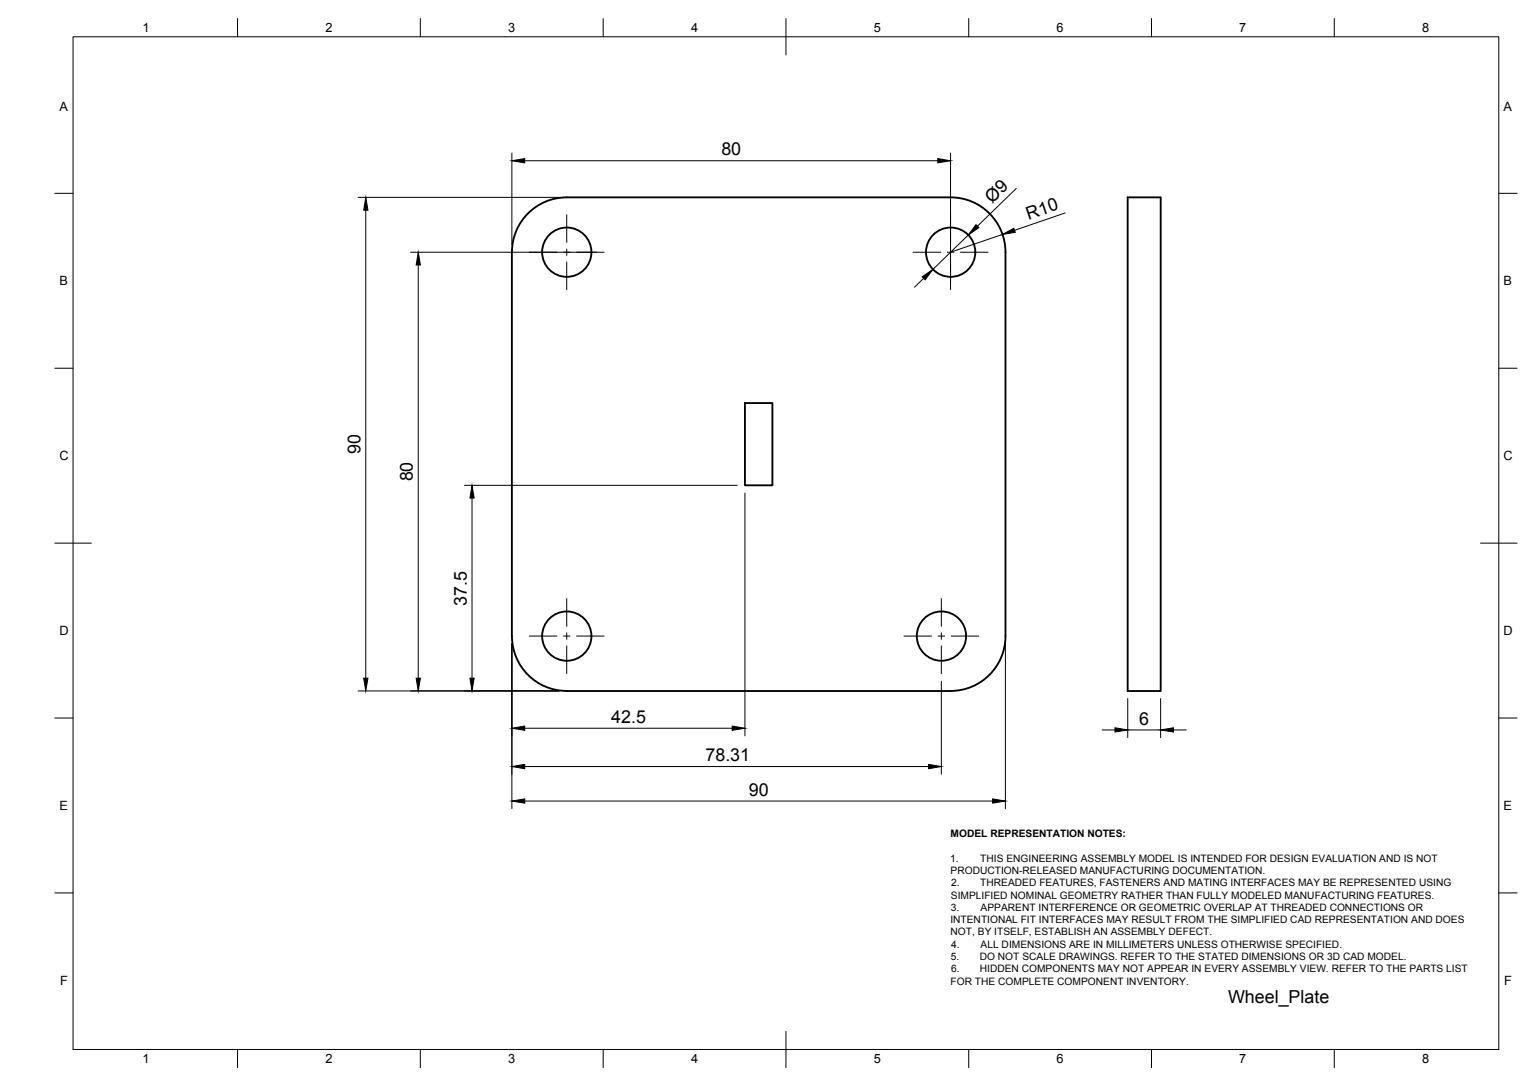
ISO-10303-21;
HEADER;
/* Generated by software containing ST-Developer
 * from STEP Tools, Inc. (www.steptools.com) 
 */

FILE_DESCRIPTION(
/* description */ ('Wheel Holder-Mirrored'),
/* implementation_level */ '2;1');

FILE_NAME(
/* name */ 'Wheel_Plate.step',
/* time_stamp */ '2026-10-07T09:01:46-07:00',
/* author */ (''),
/* organization */ (''),
/* preprocessor_version */ 'ST-DEVELOPER v20.2',
/* originating_system */ 'Autodesk Translation Framework v15.15.0.0',
/* authorisation */ '');

FILE_SCHEMA (('AUTOMOTIVE_DESIGN { 1 0 10303 214 3 1 1 }'));
ENDSEC;

DATA;
#10=MECHANICAL_DESIGN_GEOMETRIC_PRESENTATION_REPRESENTATION('',(#200),#3832);
#188=SHAPE_REPRESENTATION_RELATIONSHIP('SRR','None',#3865,#194);
#194=ADVANCED_BREP_SHAPE_REPRESENTATION('',(#206),#3828);
#200=STYLED_ITEM('',(#3904),#206);
#206=MANIFOLD_SOLID_BREP('Body1',#1785);
#214=FACE_BOUND('',#393,.T.);
#215=FACE_BOUND('',#394,.T.);
#216=FACE_BOUND('',#395,.T.);
#217=FACE_BOUND('',#396,.T.);
#218=FACE_BOUND('',#397,.T.);
#219=FACE_BOUND('',#399,.T.);
#220=FACE_BOUND('',#400,.T.);
#221=FACE_BOUND('',#401,.T.);
#222=FACE_BOUND('',#402,.T.);
#223=FACE_BOUND('',#403,.T.);
#233=PLANE('',#1881);
#234=PLANE('',#1890);
#235=PLANE('',#1899);
#236=PLANE('',#1901);
#237=PLANE('',#1903);
#238=PLANE('',#1905);
#239=PLANE('',#1911);
#240=PLANE('',#1912);
#241=PLANE('',#1913);
#242=PLANE('',#1914);
#284=FACE_OUTER_BOUND('',#392,.T.);
#285=FACE_OUTER_BOUND('',#398,.T.);
#286=FACE_OUTER_BOUND('',#404,.T.);
#287=FACE_OUTER_BOUND('',#405,.T.);
#288=FACE_OUTER_BOUND('',#406,.T.);
#289=FACE_OUTER_BOUND('',#407,.T.);
#290=FACE_OUTER_BOUND('',#408,.T.);
#291=FACE_OUTER_BOUND('',#409,.T.);
#292=FACE_OUTER_BOUND('',#410,.T.);
#293=FACE_OUTER_BOUND('',#411,.T.);
#294=FACE_OUTER_BOUND('',#412,.T.);
#295=FACE_OUTER_BOUND('',#413,.T.);
#296=FACE_OUTER_BOUND('',#414,.T.);
#297=FACE_OUTER_BOUND('',#415,.T.);
#298=FACE_OUTER_BOUND('',#416,.T.);
#299=FACE_OUTER_BOUND('',#417,.T.);
#300=FACE_OUTER_BOUND('',#418,.T.);
#301=FACE_OUTER_BOUND('',#419,.T.);
#392=EDGE_LOOP('',(#1183,#1184,#1185,#1186,#1187,#1188,#1189,#1190));
#393=EDGE_LOOP('',(#1191,#1192,#1193,#1194));
#394=EDGE_LOOP('',(#1195));
#395=EDGE_LOOP('',(#1196));
#396=EDGE_LOOP('',(#1197));
#397=EDGE_LOOP('',(#1198));
#398=EDGE_LOOP('',(#1199,#1200,#1201,#1202,#1203,#1204,#1205,#1206));
#399=EDGE_LOOP('',(#1207));
#400=EDGE_LOOP('',(#1208));
#401=EDGE_LOOP('',(#1209));
#402=EDGE_LOOP('',(#1210));
#403=EDGE_LOOP('',(#1211,#1212,#1213,#1214));
#404=EDGE_LOOP('',(#1215,#1216,#1217,#1218));
#405=EDGE_LOOP('',(#1219,#1220,#1221,#1222));
#406=EDGE_LOOP('',(#1223,#1224,#1225,#1226));
#407=EDGE_LOOP('',(#1227,#1228,#1229,#1230));
#408=EDGE_LOOP('',(#1231,#1232,#1233,#1234));
#409=EDGE_LOOP('',(#1235,#1236,#1237,#1238));
#410=EDGE_LOOP('',(#1239,#1240,#1241,#1242));
#411=EDGE_LOOP('',(#1243,#1244,#1245,#1246));
#412=EDGE_LOOP('',(#1247,#1248,#1249,#1250));
#413=EDGE_LOOP('',(#1251,#1252,#1253,#1254));
#414=EDGE_LOOP('',(#1255,#1256,#1257,#1258));
#415=EDGE_LOOP('',(#1259,#1260,#1261,#1262));
#416=EDGE_LOOP('',(#1263,#1264,#1265,#1266));
#417=EDGE_LOOP('',(#1267,#1268,#1269,#1270));
#418=EDGE_LOOP('',(#1271,#1272,#1273,#1274));
#419=EDGE_LOOP('',(#1275,#1276,#1277,#1278));
#503=LINE('',#2568,#596);
#504=LINE('',#2572,#597);
#505=LINE('',#2576,#598);
#506=LINE('',#2580,#599);
#507=LINE('',#2584,#600);
#508=LINE('',#2586,#601);
#509=LINE('',#2588,#602);
#510=LINE('',#2589,#603);
#511=LINE('',#2601,#604);
#512=LINE('',#2605,#605);
#513=LINE('',#2609,#606);
#514=LINE('',#2613,#607);
#515=LINE('',#2625,#608);
#516=LINE('',#2627,#609);
#517=LINE('',#2629,#610);
#518=LINE('',#2630,#611);
#519=LINE('',#2632,#612);
#520=LINE('',#2633,#613);
#521=LINE('',#2635,#614);
#522=LINE('',#2637,#615);
#523=LINE('',#2639,#616);
#524=LINE('',#2641,#617);
#525=LINE('',#2643,#618);
#526=LINE('',#2645,#619);
#527=LINE('',#2647,#620);
#528=LINE('',#2649,#621);
#529=LINE('',#2651,#622);
#530=LINE('',#2653,#623);
#531=LINE('',#2656,#624);
#532=LINE('',#2657,#625);
#533=LINE('',#2659,#626);
#534=LINE('',#2661,#627);
#596=VECTOR('',#2105,1.);
#597=VECTOR('',#2108,1.);
#598=VECTOR('',#2111,1.);
#599=VECTOR('',#2114,1.);
#600=VECTOR('',#2117,1.);
#601=VECTOR('',#2118,1.);
#602=VECTOR('',#2119,1.);
#603=VECTOR('',#2120,1.);
#604=VECTOR('',#2131,1.);
#605=VECTOR('',#2134,1.);
#606=VECTOR('',#2137,1.);
#607=VECTOR('',#2140,1.);
#608=VECTOR('',#2151,1.);
#609=VECTOR('',#2152,1.);
#610=VECTOR('',#2153,1.);
#611=VECTOR('',#2154,1.);
#612=VECTOR('',#2157,1.);
#613=VECTOR('',#2158,1.);
#614=VECTOR('',#2161,1.);
#615=VECTOR('',#2164,1.);
#616=VECTOR('',#2167,1.);
#617=VECTOR('',#2170,1.);
#618=VECTOR('',#2173,1.);
#619=VECTOR('',#2176,1.);
#620=VECTOR('',#2179,0.0045);
#621=VECTOR('',#2182,0.0045);
#622=VECTOR('',#2185,0.0045);
#623=VECTOR('',#2188,0.0045);
#624=VECTOR('',#2193,1.);
#625=VECTOR('',#2194,1.);
#626=VECTOR('',#2197,1.);
#627=VECTOR('',#2200,1.);
#694=CIRCLE('',#1882,0.01);
#695=CIRCLE('',#1883,0.0100000000000001);
#696=CIRCLE('',#1884,0.0100000000000001);
#697=CIRCLE('',#1885,0.01);
#698=CIRCLE('',#1886,0.0045);
#699=CIRCLE('',#1887,0.0045);
#700=CIRCLE('',#1888,0.0045);
#701=CIRCLE('',#1889,0.0045);
#702=CIRCLE('',#1891,0.01);
#703=CIRCLE('',#1892,0.0100000000000001);
#704=CIRCLE('',#1893,0.0100000000000001);
#705=CIRCLE('',#1894,0.01);
#706=CIRCLE('',#1895,0.0045);
#707=CIRCLE('',#1896,0.0045);
#708=CIRCLE('',#1897,0.0045);
#709=CIRCLE('',#1898,0.0045);
#756=VERTEX_POINT('',#2566);
#757=VERTEX_POINT('',#2567);
#758=VERTEX_POINT('',#2569);
#759=VERTEX_POINT('',#2571);
#760=VERTEX_POINT('',#2573);
#761=VERTEX_POINT('',#2575);
#762=VERTEX_POINT('',#2577);
#763=VERTEX_POINT('',#2579);
#764=VERTEX_POINT('',#2582);
#765=VERTEX_POINT('',#2583);
#766=VERTEX_POINT('',#2585);
#767=VERTEX_POINT('',#2587);
#768=VERTEX_POINT('',#2590);
#769=VERTEX_POINT('',#2592);
#770=VERTEX_POINT('',#2594);
#771=VERTEX_POINT('',#2596);
#772=VERTEX_POINT('',#2599);
#773=VERTEX_POINT('',#2600);
#774=VERTEX_POINT('',#2602);
#775=VERTEX_POINT('',#2604);
#776=VERTEX_POINT('',#2606);
#777=VERTEX_POINT('',#2608);
#778=VERTEX_POINT('',#2610);
#779=VERTEX_POINT('',#2612);
#780=VERTEX_POINT('',#2615);
#781=VERTEX_POINT('',#2617);
#782=VERTEX_POINT('',#2619);
#783=VERTEX_POINT('',#2621);
#784=VERTEX_POINT('',#2623);
#785=VERTEX_POINT('',#2624);
#786=VERTEX_POINT('',#2626);
#787=VERTEX_POINT('',#2628);
#918=EDGE_CURVE('',#756,#757,#503,.T.);
#919=EDGE_CURVE('',#758,#756,#694,.T.);
#920=EDGE_CURVE('',#758,#759,#504,.T.);
#921=EDGE_CURVE('',#760,#759,#695,.T.);
#922=EDGE_CURVE('',#760,#761,#505,.T.);
#923=EDGE_CURVE('',#762,#761,#696,.T.);
#924=EDGE_CURVE('',#763,#762,#506,.T.);
#925=EDGE_CURVE('',#757,#763,#697,.T.);
#926=EDGE_CURVE('',#764,#765,#507,.T.);
#927=EDGE_CURVE('',#765,#766,#508,.T.);
#928=EDGE_CURVE('',#767,#766,#509,.T.);
#929=EDGE_CURVE('',#764,#767,#510,.T.);
#930=EDGE_CURVE('',#768,#768,#698,.T.);
#931=EDGE_CURVE('',#769,#769,#699,.T.);
#932=EDGE_CURVE('',#770,#770,#700,.T.);
#933=EDGE_CURVE('',#771,#771,#701,.T.);
#934=EDGE_CURVE('',#772,#773,#511,.T.);
#935=EDGE_CURVE('',#773,#774,#702,.T.);
#936=EDGE_CURVE('',#774,#775,#512,.T.);
#937=EDGE_CURVE('',#775,#776,#703,.T.);
#938=EDGE_CURVE('',#777,#776,#513,.T.);
#939=EDGE_CURVE('',#777,#778,#704,.T.);
#940=EDGE_CURVE('',#779,#778,#514,.T.);
#941=EDGE_CURVE('',#779,#772,#705,.T.);
#942=EDGE_CURVE('',#780,#780,#706,.T.);
#943=EDGE_CURVE('',#781,#781,#707,.T.);
#944=EDGE_CURVE('',#782,#782,#708,.T.);
#945=EDGE_CURVE('',#783,#783,#709,.T.);
#946=EDGE_CURVE('',#784,#785,#515,.T.);
#947=EDGE_CURVE('',#786,#784,#516,.T.);
#948=EDGE_CURVE('',#786,#787,#517,.T.);
#949=EDGE_CURVE('',#787,#785,#518,.T.);
#950=EDGE_CURVE('',#756,#772,#519,.T.);
#951=EDGE_CURVE('',#757,#773,#520,.T.);
#952=EDGE_CURVE('',#763,#774,#521,.T.);
#953=EDGE_CURVE('',#762,#775,#522,.T.);
#954=EDGE_CURVE('',#761,#776,#523,.T.);
#955=EDGE_CURVE('',#760,#777,#524,.T.);
#956=EDGE_CURVE('',#759,#778,#525,.T.);
#957=EDGE_CURVE('',#758,#779,#526,.T.);
#958=EDGE_CURVE('',#771,#780,#527,.T.);
#959=EDGE_CURVE('',#770,#781,#528,.T.);
#960=EDGE_CURVE('',#769,#782,#529,.T.);
#961=EDGE_CURVE('',#768,#783,#530,.T.);
#962=EDGE_CURVE('',#765,#784,#531,.T.);
#963=EDGE_CURVE('',#766,#785,#532,.T.);
#964=EDGE_CURVE('',#767,#787,#533,.T.);
#965=EDGE_CURVE('',#764,#786,#534,.T.);
#1183=ORIENTED_EDGE('',*,*,#918,.F.);
#1184=ORIENTED_EDGE('',*,*,#919,.F.);
#1185=ORIENTED_EDGE('',*,*,#920,.T.);
#1186=ORIENTED_EDGE('',*,*,#921,.F.);
#1187=ORIENTED_EDGE('',*,*,#922,.T.);
#1188=ORIENTED_EDGE('',*,*,#923,.F.);
#1189=ORIENTED_EDGE('',*,*,#924,.F.);
#1190=ORIENTED_EDGE('',*,*,#925,.F.);
#1191=ORIENTED_EDGE('',*,*,#926,.T.);
#1192=ORIENTED_EDGE('',*,*,#927,.T.);
#1193=ORIENTED_EDGE('',*,*,#928,.F.);
#1194=ORIENTED_EDGE('',*,*,#929,.F.);
#1195=ORIENTED_EDGE('',*,*,#930,.T.);
#1196=ORIENTED_EDGE('',*,*,#931,.T.);
#1197=ORIENTED_EDGE('',*,*,#932,.T.);
#1198=ORIENTED_EDGE('',*,*,#933,.T.);
#1199=ORIENTED_EDGE('',*,*,#934,.T.);
#1200=ORIENTED_EDGE('',*,*,#935,.T.);
#1201=ORIENTED_EDGE('',*,*,#936,.T.);
#1202=ORIENTED_EDGE('',*,*,#937,.T.);
#1203=ORIENTED_EDGE('',*,*,#938,.F.);
#1204=ORIENTED_EDGE('',*,*,#939,.T.);
#1205=ORIENTED_EDGE('',*,*,#940,.F.);
#1206=ORIENTED_EDGE('',*,*,#941,.T.);
#1207=ORIENTED_EDGE('',*,*,#942,.F.);
#1208=ORIENTED_EDGE('',*,*,#943,.F.);
#1209=ORIENTED_EDGE('',*,*,#944,.F.);
#1210=ORIENTED_EDGE('',*,*,#945,.F.);
#1211=ORIENTED_EDGE('',*,*,#946,.F.);
#1212=ORIENTED_EDGE('',*,*,#947,.F.);
#1213=ORIENTED_EDGE('',*,*,#948,.T.);
#1214=ORIENTED_EDGE('',*,*,#949,.T.);
#1215=ORIENTED_EDGE('',*,*,#934,.F.);
#1216=ORIENTED_EDGE('',*,*,#950,.F.);
#1217=ORIENTED_EDGE('',*,*,#918,.T.);
#1218=ORIENTED_EDGE('',*,*,#951,.T.);
#1219=ORIENTED_EDGE('',*,*,#935,.F.);
#1220=ORIENTED_EDGE('',*,*,#951,.F.);
#1221=ORIENTED_EDGE('',*,*,#925,.T.);
#1222=ORIENTED_EDGE('',*,*,#952,.T.);
#1223=ORIENTED_EDGE('',*,*,#936,.F.);
#1224=ORIENTED_EDGE('',*,*,#952,.F.);
#1225=ORIENTED_EDGE('',*,*,#924,.T.);
#1226=ORIENTED_EDGE('',*,*,#953,.T.);
#1227=ORIENTED_EDGE('',*,*,#937,.F.);
#1228=ORIENTED_EDGE('',*,*,#953,.F.);
#1229=ORIENTED_EDGE('',*,*,#923,.T.);
#1230=ORIENTED_EDGE('',*,*,#954,.T.);
#1231=ORIENTED_EDGE('',*,*,#938,.T.);
#1232=ORIENTED_EDGE('',*,*,#954,.F.);
#1233=ORIENTED_EDGE('',*,*,#922,.F.);
#1234=ORIENTED_EDGE('',*,*,#955,.T.);
#1235=ORIENTED_EDGE('',*,*,#939,.F.);
#1236=ORIENTED_EDGE('',*,*,#955,.F.);
#1237=ORIENTED_EDGE('',*,*,#921,.T.);
#1238=ORIENTED_EDGE('',*,*,#956,.T.);
#1239=ORIENTED_EDGE('',*,*,#940,.T.);
#1240=ORIENTED_EDGE('',*,*,#956,.F.);
#1241=ORIENTED_EDGE('',*,*,#920,.F.);
#1242=ORIENTED_EDGE('',*,*,#957,.T.);
#1243=ORIENTED_EDGE('',*,*,#933,.F.);
#1244=ORIENTED_EDGE('',*,*,#958,.T.);
#1245=ORIENTED_EDGE('',*,*,#942,.T.);
#1246=ORIENTED_EDGE('',*,*,#958,.F.);
#1247=ORIENTED_EDGE('',*,*,#932,.F.);
#1248=ORIENTED_EDGE('',*,*,#959,.T.);
#1249=ORIENTED_EDGE('',*,*,#943,.T.);
#1250=ORIENTED_EDGE('',*,*,#959,.F.);
#1251=ORIENTED_EDGE('',*,*,#931,.F.);
#1252=ORIENTED_EDGE('',*,*,#960,.T.);
#1253=ORIENTED_EDGE('',*,*,#944,.T.);
#1254=ORIENTED_EDGE('',*,*,#960,.F.);
#1255=ORIENTED_EDGE('',*,*,#930,.F.);
#1256=ORIENTED_EDGE('',*,*,#961,.T.);
#1257=ORIENTED_EDGE('',*,*,#945,.T.);
#1258=ORIENTED_EDGE('',*,*,#961,.F.);
#1259=ORIENTED_EDGE('',*,*,#941,.F.);
#1260=ORIENTED_EDGE('',*,*,#957,.F.);
#1261=ORIENTED_EDGE('',*,*,#919,.T.);
#1262=ORIENTED_EDGE('',*,*,#950,.T.);
#1263=ORIENTED_EDGE('',*,*,#962,.T.);
#1264=ORIENTED_EDGE('',*,*,#946,.T.);
#1265=ORIENTED_EDGE('',*,*,#963,.F.);
#1266=ORIENTED_EDGE('',*,*,#927,.F.);
#1267=ORIENTED_EDGE('',*,*,#928,.T.);
#1268=ORIENTED_EDGE('',*,*,#963,.T.);
#1269=ORIENTED_EDGE('',*,*,#949,.F.);
#1270=ORIENTED_EDGE('',*,*,#964,.F.);
#1271=ORIENTED_EDGE('',*,*,#929,.T.);
#1272=ORIENTED_EDGE('',*,*,#964,.T.);
#1273=ORIENTED_EDGE('',*,*,#948,.F.);
#1274=ORIENTED_EDGE('',*,*,#965,.F.);
#1275=ORIENTED_EDGE('',*,*,#965,.T.);
#1276=ORIENTED_EDGE('',*,*,#947,.T.);
#1277=ORIENTED_EDGE('',*,*,#962,.F.);
#1278=ORIENTED_EDGE('',*,*,#926,.F.);
#1658=CYLINDRICAL_SURFACE('',#1900,0.01);
#1659=CYLINDRICAL_SURFACE('',#1902,0.0100000000000001);
#1660=CYLINDRICAL_SURFACE('',#1904,0.0100000000000001);
#1661=CYLINDRICAL_SURFACE('',#1906,0.0045);
#1662=CYLINDRICAL_SURFACE('',#1907,0.0045);
#1663=CYLINDRICAL_SURFACE('',#1908,0.0045);
#1664=CYLINDRICAL_SURFACE('',#1909,0.0045);
#1665=CYLINDRICAL_SURFACE('',#1910,0.01);
#1690=ADVANCED_FACE('',(#284,#214,#215,#216,#217,#218),#233,.T.);
#1691=ADVANCED_FACE('',(#285,#219,#220,#221,#222,#223),#234,.F.);
#1692=ADVANCED_FACE('',(#286),#235,.F.);
#1693=ADVANCED_FACE('',(#287),#1658,.T.);
#1694=ADVANCED_FACE('',(#288),#236,.F.);
#1695=ADVANCED_FACE('',(#289),#1659,.T.);
#1696=ADVANCED_FACE('',(#290),#237,.T.);
#1697=ADVANCED_FACE('',(#291),#1660,.T.);
#1698=ADVANCED_FACE('',(#292),#238,.T.);
#1699=ADVANCED_FACE('',(#293),#1661,.F.);
#1700=ADVANCED_FACE('',(#294),#1662,.F.);
#1701=ADVANCED_FACE('',(#295),#1663,.F.);
#1702=ADVANCED_FACE('',(#296),#1664,.F.);
#1703=ADVANCED_FACE('',(#297),#1665,.T.);
#1704=ADVANCED_FACE('',(#298),#239,.T.);
#1705=ADVANCED_FACE('',(#299),#240,.F.);
#1706=ADVANCED_FACE('',(#300),#241,.F.);
#1707=ADVANCED_FACE('',(#301),#242,.T.);
#1785=CLOSED_SHELL('',(#1690,#1691,#1692,#1693,#1694,#1695,#1696,#1697,
#1698,#1699,#1700,#1701,#1702,#1703,#1704,#1705,#1706,#1707));
#1880=AXIS2_PLACEMENT_3D('',#2564,#2101,#2102);
#1881=AXIS2_PLACEMENT_3D('',#2565,#2103,#2104);
#1882=AXIS2_PLACEMENT_3D('',#2570,#2106,#2107);
#1883=AXIS2_PLACEMENT_3D('',#2574,#2109,#2110);
#1884=AXIS2_PLACEMENT_3D('',#2578,#2112,#2113);
#1885=AXIS2_PLACEMENT_3D('',#2581,#2115,#2116);
#1886=AXIS2_PLACEMENT_3D('',#2591,#2121,#2122);
#1887=AXIS2_PLACEMENT_3D('',#2593,#2123,#2124);
#1888=AXIS2_PLACEMENT_3D('',#2595,#2125,#2126);
#1889=AXIS2_PLACEMENT_3D('',#2597,#2127,#2128);
#1890=AXIS2_PLACEMENT_3D('',#2598,#2129,#2130);
#1891=AXIS2_PLACEMENT_3D('',#2603,#2132,#2133);
#1892=AXIS2_PLACEMENT_3D('',#2607,#2135,#2136);
#1893=AXIS2_PLACEMENT_3D('',#2611,#2138,#2139);
#1894=AXIS2_PLACEMENT_3D('',#2614,#2141,#2142);
#1895=AXIS2_PLACEMENT_3D('',#2616,#2143,#2144);
#1896=AXIS2_PLACEMENT_3D('',#2618,#2145,#2146);
#1897=AXIS2_PLACEMENT_3D('',#2620,#2147,#2148);
#1898=AXIS2_PLACEMENT_3D('',#2622,#2149,#2150);
#1899=AXIS2_PLACEMENT_3D('',#2631,#2155,#2156);
#1900=AXIS2_PLACEMENT_3D('',#2634,#2159,#2160);
#1901=AXIS2_PLACEMENT_3D('',#2636,#2162,#2163);
#1902=AXIS2_PLACEMENT_3D('',#2638,#2165,#2166);
#1903=AXIS2_PLACEMENT_3D('',#2640,#2168,#2169);
#1904=AXIS2_PLACEMENT_3D('',#2642,#2171,#2172);
#1905=AXIS2_PLACEMENT_3D('',#2644,#2174,#2175);
#1906=AXIS2_PLACEMENT_3D('',#2646,#2177,#2178);
#1907=AXIS2_PLACEMENT_3D('',#2648,#2180,#2181);
#1908=AXIS2_PLACEMENT_3D('',#2650,#2183,#2184);
#1909=AXIS2_PLACEMENT_3D('',#2652,#2186,#2187);
#1910=AXIS2_PLACEMENT_3D('',#2654,#2189,#2190);
#1911=AXIS2_PLACEMENT_3D('',#2655,#2191,#2192);
#1912=AXIS2_PLACEMENT_3D('',#2658,#2195,#2196);
#1913=AXIS2_PLACEMENT_3D('',#2660,#2198,#2199);
#1914=AXIS2_PLACEMENT_3D('',#2662,#2201,#2202);
#2101=DIRECTION('axis',(0.,0.,1.));
#2102=DIRECTION('refdir',(1.,0.,0.));
#2103=DIRECTION('center_axis',(-4.62592926927149E-16,-2.83256473634769E-32,
-1.));
#2104=DIRECTION('ref_axis',(-1.,1.3103244120977E-47,4.62592926927149E-16));
#2105=DIRECTION('',(1.3103244120977E-47,-1.,2.83256473634769E-32));
#2106=DIRECTION('center_axis',(4.62592926927149E-16,2.83256473634769E-32,
1.));
#2107=DIRECTION('ref_axis',(1.,-7.59501135632552E-64,-4.62592926927149E-16));
#2108=DIRECTION('',(1.,-4.67973004320639E-49,-4.62592926927149E-16));
#2109=DIRECTION('center_axis',(4.62592926927149E-16,2.83256473634769E-32,
1.));
#2110=DIRECTION('ref_axis',(1.,-7.59501135632553E-64,-4.62592926927149E-16));
#2111=DIRECTION('',(1.3103244120977E-47,-1.,2.83256473634769E-32));
#2112=DIRECTION('center_axis',(4.62592926927149E-16,2.83256473634769E-32,
1.));
#2113=DIRECTION('ref_axis',(1.,-7.59501135632553E-64,-4.62592926927149E-16));
#2114=DIRECTION('',(1.,-4.67973004320639E-49,-4.62592926927149E-16));
#2115=DIRECTION('center_axis',(4.62592926927149E-16,2.83256473634769E-32,
1.));
#2116=DIRECTION('ref_axis',(1.,-7.59501135632552E-64,-4.62592926927149E-16));
#2117=DIRECTION('',(1.3103244120977E-47,-1.,2.83256473634769E-32));
#2118=DIRECTION('',(1.,-1.3103244120977E-47,-4.62592926927149E-16));
#2119=DIRECTION('',(1.3103244120977E-47,-1.,2.83256473634769E-32));
#2120=DIRECTION('',(1.,-1.3103244120977E-47,-4.62592926927149E-16));
#2121=DIRECTION('center_axis',(4.62592926927149E-16,2.83256473634769E-32,
1.));
#2122=DIRECTION('ref_axis',(1.,-7.59501135632552E-64,-4.62592926927149E-16));
#2123=DIRECTION('center_axis',(4.62592926927149E-16,2.83256473634769E-32,
1.));
#2124=DIRECTION('ref_axis',(1.,-7.59501135632552E-64,-4.62592926927149E-16));
#2125=DIRECTION('center_axis',(4.62592926927149E-16,2.83256473634769E-32,
1.));
#2126=DIRECTION('ref_axis',(1.,-7.59501135632552E-64,-4.62592926927149E-16));
#2127=DIRECTION('center_axis',(4.62592926927149E-16,2.83256473634769E-32,
1.));
#2128=DIRECTION('ref_axis',(1.,-7.59501135632552E-64,-4.62592926927149E-16));
#2129=DIRECTION('center_axis',(-4.62592926927149E-16,-2.83256473634769E-32,
-1.));
#2130=DIRECTION('ref_axis',(-1.,1.3103244120977E-47,4.62592926927149E-16));
#2131=DIRECTION('',(1.3103244120977E-47,-1.,2.83256473634769E-32));
#2132=DIRECTION('center_axis',(4.62592926927149E-16,2.83256473634769E-32,
1.));
#2133=DIRECTION('ref_axis',(1.,-7.59501135632552E-64,-4.62592926927149E-16));
#2134=DIRECTION('',(1.,-4.67973004320639E-49,-4.62592926927149E-16));
#2135=DIRECTION('center_axis',(4.62592926927149E-16,2.83256473634769E-32,
1.));
#2136=DIRECTION('ref_axis',(1.,-7.59501135632553E-64,-4.62592926927149E-16));
#2137=DIRECTION('',(1.3103244120977E-47,-1.,2.83256473634769E-32));
#2138=DIRECTION('center_axis',(4.62592926927149E-16,2.83256473634769E-32,
1.));
#2139=DIRECTION('ref_axis',(1.,-7.59501135632553E-64,-4.62592926927149E-16));
#2140=DIRECTION('',(1.,-4.67973004320639E-49,-4.62592926927149E-16));
#2141=DIRECTION('center_axis',(4.62592926927149E-16,2.83256473634769E-32,
1.));
#2142=DIRECTION('ref_axis',(1.,-7.59501135632552E-64,-4.62592926927149E-16));
#2143=DIRECTION('center_axis',(4.62592926927149E-16,2.83256473634769E-32,
1.));
#2144=DIRECTION('ref_axis',(1.,-7.59501135632552E-64,-4.62592926927149E-16));
#2145=DIRECTION('center_axis',(4.62592926927149E-16,2.83256473634769E-32,
1.));
#2146=DIRECTION('ref_axis',(1.,-7.59501135632552E-64,-4.62592926927149E-16));
#2147=DIRECTION('center_axis',(4.62592926927149E-16,2.83256473634769E-32,
1.));
#2148=DIRECTION('ref_axis',(1.,-7.59501135632552E-64,-4.62592926927149E-16));
#2149=DIRECTION('center_axis',(4.62592926927149E-16,2.83256473634769E-32,
1.));
#2150=DIRECTION('ref_axis',(1.,-7.59501135632552E-64,-4.62592926927149E-16));
#2151=DIRECTION('',(1.,-1.3103244120977E-47,-4.62592926927149E-16));
#2152=DIRECTION('',(1.3103244120977E-47,-1.,2.83256473634769E-32));
#2153=DIRECTION('',(1.,-1.3103244120977E-47,-4.62592926927149E-16));
#2154=DIRECTION('',(1.3103244120977E-47,-1.,2.83256473634769E-32));
#2155=DIRECTION('center_axis',(1.,0.,-4.62592926927149E-16));
#2156=DIRECTION('ref_axis',(4.62592926927149E-16,0.,1.));
#2157=DIRECTION('',(4.62592926927149E-16,2.83256473634769E-32,1.));
#2158=DIRECTION('',(4.62592926927149E-16,2.83256473634769E-32,1.));
#2159=DIRECTION('center_axis',(4.62592926927149E-16,2.83256473634769E-32,
1.));
#2160=DIRECTION('ref_axis',(-1.,7.59501135632552E-64,4.62592926927149E-16));
#2161=DIRECTION('',(4.62592926927149E-16,2.83256473634769E-32,1.));
#2162=DIRECTION('center_axis',(-1.26352711166564E-47,1.,-2.83256473634769E-32));
#2163=DIRECTION('ref_axis',(2.23962894278238E-95,2.83256473634769E-32,1.));
#2164=DIRECTION('',(4.62592926927149E-16,2.83256473634769E-32,1.));
#2165=DIRECTION('center_axis',(4.62592926927149E-16,2.83256473634769E-32,
1.));
#2166=DIRECTION('ref_axis',(-1.,7.59501135632553E-64,4.62592926927149E-16));
#2167=DIRECTION('',(4.62592926927149E-16,2.83256473634769E-32,1.));
#2168=DIRECTION('center_axis',(1.,0.,-4.62592926927149E-16));
#2169=DIRECTION('ref_axis',(4.62592926927149E-16,0.,1.));
#2170=DIRECTION('',(4.62592926927149E-16,2.83256473634769E-32,1.));
#2171=DIRECTION('center_axis',(4.62592926927149E-16,2.83256473634769E-32,
1.));
#2172=DIRECTION('ref_axis',(-1.,7.59501135632553E-64,4.62592926927149E-16));
#2173=DIRECTION('',(4.62592926927149E-16,2.83256473634769E-32,1.));
#2174=DIRECTION('center_axis',(-1.26352711166564E-47,1.,-2.83256473634769E-32));
#2175=DIRECTION('ref_axis',(2.23962894278238E-95,2.83256473634769E-32,1.));
#2176=DIRECTION('',(4.62592926927149E-16,2.83256473634769E-32,1.));
#2177=DIRECTION('center_axis',(4.62592926927149E-16,2.83256473634769E-32,
1.));
#2178=DIRECTION('ref_axis',(-1.,7.59501135632552E-64,4.62592926927149E-16));
#2179=DIRECTION('',(4.62592926927149E-16,2.83256473634769E-32,1.));
#2180=DIRECTION('center_axis',(4.62592926927149E-16,2.83256473634769E-32,
1.));
#2181=DIRECTION('ref_axis',(-1.,7.59501135632552E-64,4.62592926927149E-16));
#2182=DIRECTION('',(4.62592926927149E-16,2.83256473634769E-32,1.));
#2183=DIRECTION('center_axis',(4.62592926927149E-16,2.83256473634769E-32,
1.));
#2184=DIRECTION('ref_axis',(-1.,7.59501135632552E-64,4.62592926927149E-16));
#2185=DIRECTION('',(4.62592926927149E-16,2.83256473634769E-32,1.));
#2186=DIRECTION('center_axis',(4.62592926927149E-16,2.83256473634769E-32,
1.));
#2187=DIRECTION('ref_axis',(-1.,7.59501135632552E-64,4.62592926927149E-16));
#2188=DIRECTION('',(4.62592926927149E-16,2.83256473634769E-32,1.));
#2189=DIRECTION('center_axis',(4.62592926927149E-16,2.83256473634769E-32,
1.));
#2190=DIRECTION('ref_axis',(-1.,7.59501135632552E-64,4.62592926927149E-16));
#2191=DIRECTION('center_axis',(0.,1.,-2.83256473634769E-32));
#2192=DIRECTION('ref_axis',(0.,2.83256473634769E-32,1.));
#2193=DIRECTION('',(4.62592926927149E-16,2.83256473634769E-32,1.));
#2194=DIRECTION('',(4.62592926927149E-16,2.83256473634769E-32,1.));
#2195=DIRECTION('center_axis',(1.,0.,-4.62592926927149E-16));
#2196=DIRECTION('ref_axis',(-4.62592926927149E-16,0.,-1.));
#2197=DIRECTION('',(4.62592926927149E-16,2.83256473634769E-32,1.));
#2198=DIRECTION('center_axis',(0.,1.,-2.83256473634769E-32));
#2199=DIRECTION('ref_axis',(0.,2.83256473634769E-32,1.));
#2200=DIRECTION('',(4.62592926927149E-16,2.83256473634769E-32,1.));
#2201=DIRECTION('center_axis',(1.,0.,-4.62592926927149E-16));
#2202=DIRECTION('ref_axis',(-4.62592926927149E-16,0.,-1.));
#2564=CARTESIAN_POINT('',(0.,0.,0.));
#2565=CARTESIAN_POINT('Origin',(0.45,-0.85,-0.031));
#2566=CARTESIAN_POINT('',(0.405,-0.815,-0.031));
#2567=CARTESIAN_POINT('',(0.405,-0.885,-0.031));
#2568=CARTESIAN_POINT('',(0.405,-0.85,-0.031));
#2569=CARTESIAN_POINT('',(0.415,-0.805,-0.031));
#2570=CARTESIAN_POINT('Origin',(0.415,-0.815,-0.031));
#2571=CARTESIAN_POINT('',(0.485,-0.805,-0.031));
#2572=CARTESIAN_POINT('',(0.45,-0.805,-0.031));
#2573=CARTESIAN_POINT('',(0.495,-0.815,-0.031));
#2574=CARTESIAN_POINT('Origin',(0.485,-0.815,-0.031));
#2575=CARTESIAN_POINT('',(0.495,-0.885,-0.031));
#2576=CARTESIAN_POINT('',(0.495,-0.85,-0.031));
#2577=CARTESIAN_POINT('',(0.485,-0.895,-0.031));
#2578=CARTESIAN_POINT('Origin',(0.485,-0.885,-0.031));
#2579=CARTESIAN_POINT('',(0.415,-0.895,-0.031));
#2580=CARTESIAN_POINT('',(0.45,-0.895,-0.031));
#2581=CARTESIAN_POINT('Origin',(0.415,-0.885,-0.031));
#2582=CARTESIAN_POINT('',(0.4475,-0.8425,-0.031));
#2583=CARTESIAN_POINT('',(0.4475,-0.8575,-0.031));
#2584=CARTESIAN_POINT('',(0.4475,-0.85,-0.031));
#2585=CARTESIAN_POINT('',(0.4525,-0.8575,-0.031));
#2586=CARTESIAN_POINT('',(0.45,-0.8575,-0.031));
#2587=CARTESIAN_POINT('',(0.4525,-0.8425,-0.031));
#2588=CARTESIAN_POINT('',(0.4525,-0.85,-0.031));
#2589=CARTESIAN_POINT('',(0.45,-0.8425,-0.031));
#2590=CARTESIAN_POINT('',(0.4195,-0.885,-0.031));
#2591=CARTESIAN_POINT('Origin',(0.415,-0.885,-0.031));
#2592=CARTESIAN_POINT('',(0.421185503721238,-0.815,-0.031));
#2593=CARTESIAN_POINT('Origin',(0.416685503721238,-0.815,-0.031));
#2594=CARTESIAN_POINT('',(0.4895,-0.815,-0.031));
#2595=CARTESIAN_POINT('Origin',(0.485,-0.815,-0.031));
#2596=CARTESIAN_POINT('',(0.4895,-0.885,-0.031));
#2597=CARTESIAN_POINT('Origin',(0.485,-0.885,-0.031));
#2598=CARTESIAN_POINT('Origin',(0.45,-0.85,-0.025));
#2599=CARTESIAN_POINT('',(0.405,-0.815,-0.025));
#2600=CARTESIAN_POINT('',(0.405,-0.885,-0.025));
#2601=CARTESIAN_POINT('',(0.405,-0.85,-0.025));
#2602=CARTESIAN_POINT('',(0.415,-0.895,-0.025));
#2603=CARTESIAN_POINT('Origin',(0.415,-0.885,-0.025));
#2604=CARTESIAN_POINT('',(0.485,-0.895,-0.025));
#2605=CARTESIAN_POINT('',(0.45,-0.895,-0.025));
#2606=CARTESIAN_POINT('',(0.495,-0.885,-0.025));
#2607=CARTESIAN_POINT('Origin',(0.485,-0.885,-0.025));
#2608=CARTESIAN_POINT('',(0.495,-0.815,-0.025));
#2609=CARTESIAN_POINT('',(0.495,-0.85,-0.025));
#2610=CARTESIAN_POINT('',(0.485,-0.805,-0.025));
#2611=CARTESIAN_POINT('Origin',(0.485,-0.815,-0.025));
#2612=CARTESIAN_POINT('',(0.415,-0.805,-0.025));
#2613=CARTESIAN_POINT('',(0.45,-0.805,-0.025));
#2614=CARTESIAN_POINT('Origin',(0.415,-0.815,-0.025));
#2615=CARTESIAN_POINT('',(0.4895,-0.885,-0.025));
#2616=CARTESIAN_POINT('Origin',(0.485,-0.885,-0.025));
#2617=CARTESIAN_POINT('',(0.4895,-0.815,-0.025));
#2618=CARTESIAN_POINT('Origin',(0.485,-0.815,-0.025));
#2619=CARTESIAN_POINT('',(0.421185503721238,-0.815,-0.025));
#2620=CARTESIAN_POINT('Origin',(0.416685503721238,-0.815,-0.025));
#2621=CARTESIAN_POINT('',(0.4195,-0.885,-0.025));
#2622=CARTESIAN_POINT('Origin',(0.415,-0.885,-0.025));
#2623=CARTESIAN_POINT('',(0.4475,-0.8575,-0.025));
#2624=CARTESIAN_POINT('',(0.4525,-0.8575,-0.025));
#2625=CARTESIAN_POINT('',(0.45,-0.8575,-0.025));
#2626=CARTESIAN_POINT('',(0.4475,-0.8425,-0.025));
#2627=CARTESIAN_POINT('',(0.4475,-0.85,-0.025));
#2628=CARTESIAN_POINT('',(0.4525,-0.8425,-0.025));
#2629=CARTESIAN_POINT('',(0.45,-0.8425,-0.025));
#2630=CARTESIAN_POINT('',(0.4525,-0.85,-0.025));
#2631=CARTESIAN_POINT('Origin',(0.405,-0.85,-0.031));
#2632=CARTESIAN_POINT('',(0.405,-0.815,-0.031));
#2633=CARTESIAN_POINT('',(0.405,-0.885,-0.031));
#2634=CARTESIAN_POINT('Origin',(0.415,-0.885,-0.031));
#2635=CARTESIAN_POINT('',(0.415,-0.895,-0.031));
#2636=CARTESIAN_POINT('Origin',(0.45,-0.895,-0.031));
#2637=CARTESIAN_POINT('',(0.485,-0.895,-0.031));
#2638=CARTESIAN_POINT('Origin',(0.485,-0.885,-0.031));
#2639=CARTESIAN_POINT('',(0.495,-0.885,-0.031));
#2640=CARTESIAN_POINT('Origin',(0.495,-0.85,-0.031));
#2641=CARTESIAN_POINT('',(0.495,-0.815,-0.031));
#2642=CARTESIAN_POINT('Origin',(0.485,-0.815,-0.031));
#2643=CARTESIAN_POINT('',(0.485,-0.805,-0.031));
#2644=CARTESIAN_POINT('Origin',(0.45,-0.805,-0.031));
#2645=CARTESIAN_POINT('',(0.415,-0.805,-0.031));
#2646=CARTESIAN_POINT('Origin',(0.485,-0.885,-0.031));
#2647=CARTESIAN_POINT('',(0.4895,-0.885,-0.031));
#2648=CARTESIAN_POINT('Origin',(0.485,-0.815,-0.031));
#2649=CARTESIAN_POINT('',(0.4895,-0.815,-0.031));
#2650=CARTESIAN_POINT('Origin',(0.416685503721238,-0.815,-0.031));
#2651=CARTESIAN_POINT('',(0.421185503721238,-0.815,-0.031));
#2652=CARTESIAN_POINT('Origin',(0.415,-0.885,-0.031));
#2653=CARTESIAN_POINT('',(0.4195,-0.885,-0.031));
#2654=CARTESIAN_POINT('Origin',(0.415,-0.815,-0.031));
#2655=CARTESIAN_POINT('Origin',(0.45,-0.8575,-0.058));
#2656=CARTESIAN_POINT('',(0.4475,-0.8575,-0.058));
#2657=CARTESIAN_POINT('',(0.4525,-0.8575,-0.058));
#2658=CARTESIAN_POINT('Origin',(0.4525,-0.85,-0.058));
#2659=CARTESIAN_POINT('',(0.4525,-0.8425,-0.058));
#2660=CARTESIAN_POINT('Origin',(0.45,-0.8425,-0.058));
#2661=CARTESIAN_POINT('',(0.4475,-0.8425,-0.058));
#2662=CARTESIAN_POINT('Origin',(0.4475,-0.85,-0.058));
#3820=UNCERTAINTY_MEASURE_WITH_UNIT(LENGTH_MEASURE(1.E-5),#3833,
'DISTANCE_ACCURACY_VALUE',
'Maximum model space distance between geometric entities at asserted c
onnectivities');
#3824=UNCERTAINTY_MEASURE_WITH_UNIT(LENGTH_MEASURE(1.E-5),#3833,
'DISTANCE_ACCURACY_VALUE',
'Maximum model space distance between geometric entities at asserted c
onnectivities');
#3828=(
GEOMETRIC_REPRESENTATION_CONTEXT(3)
GLOBAL_UNCERTAINTY_ASSIGNED_CONTEXT((#3820))
GLOBAL_UNIT_ASSIGNED_CONTEXT((#3833,#3834,#3835))
REPRESENTATION_CONTEXT('','3D')
);
#3832=(
GEOMETRIC_REPRESENTATION_CONTEXT(3)
GLOBAL_UNCERTAINTY_ASSIGNED_CONTEXT((#3824))
GLOBAL_UNIT_ASSIGNED_CONTEXT((#3833,#3834,#3835))
REPRESENTATION_CONTEXT('','3D')
);
#3833=(
LENGTH_UNIT()
NAMED_UNIT(*)
SI_UNIT($,.METRE.)
);
#3834=(
NAMED_UNIT(*)
PLANE_ANGLE_UNIT()
SI_UNIT($,.RADIAN.)
);
#3835=(
NAMED_UNIT(*)
SI_UNIT($,.STERADIAN.)
SOLID_ANGLE_UNIT()
);
#3839=SHAPE_DEFINITION_REPRESENTATION(#3846,#3865);
#3846=PRODUCT_DEFINITION_SHAPE('',$,#3873);
#3865=SHAPE_REPRESENTATION('',(#1880),#3828);
#3869=PRODUCT_DEFINITION_CONTEXT('part definition',#3892,'design');
#3873=PRODUCT_DEFINITION('2026-10-07-15-36-10-347','Wheel_Plate',#3880,
#3869);
#3880=PRODUCT_DEFINITION_FORMATION('',$,#3897);
#3892=APPLICATION_CONTEXT(
'Core Data for Automotive Mechanical Design Process');
#3893=PRODUCT_CONTEXT('part definition',#3892,'mechanical');
#3897=PRODUCT('2026-10-07-15-36-10-347','Wheel_Plate',
'6mm-4pcs-wheel-plate',(#3893));
#3904=PRESENTATION_STYLE_ASSIGNMENT((#3910));
#3910=SURFACE_STYLE_USAGE(.BOTH.,#3916);
#3916=SURFACE_SIDE_STYLE('',(#3922));
#3922=SURFACE_STYLE_FILL_AREA(#3928);
#3928=FILL_AREA_STYLE('Opaque(157,207,237)',(#3934));
#3934=FILL_AREA_STYLE_COLOUR('Opaque(157,207,237)',#3940);
#3940=COLOUR_RGB('Opaque(157,207,237)', 0.31764706, 0.68627451, 0.89019608);
ENDSEC;
END-ISO-10303-21;
